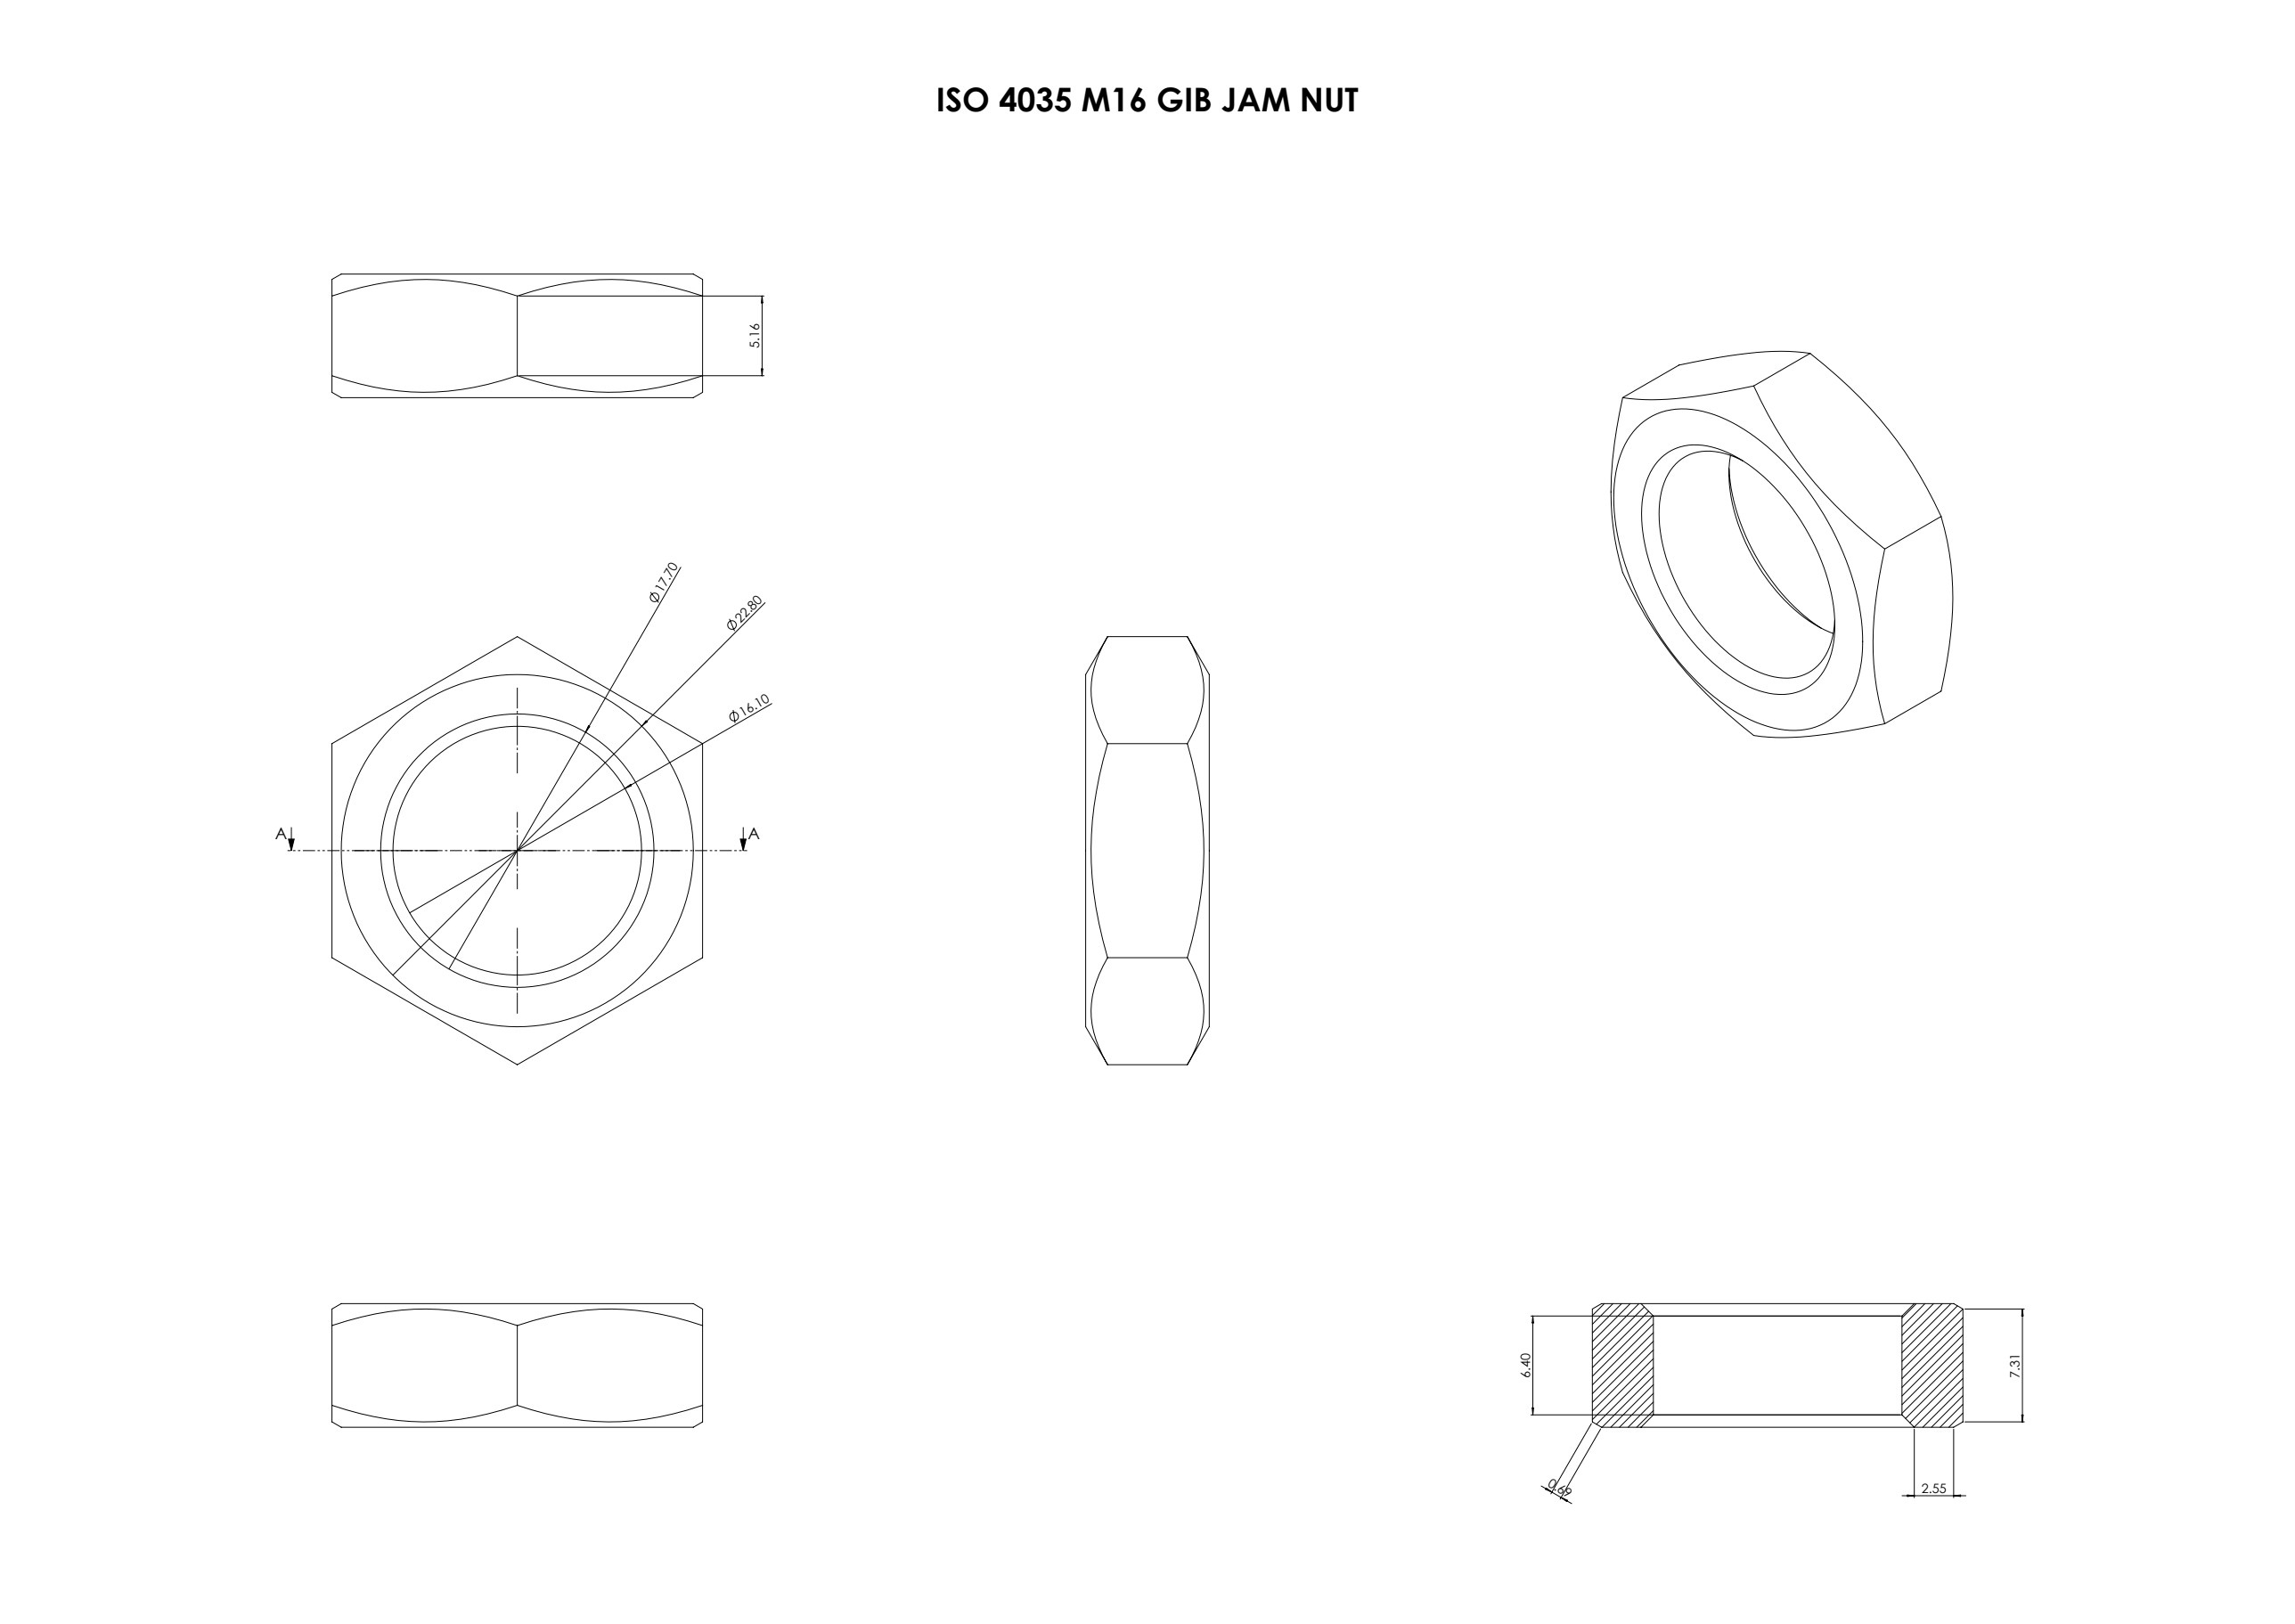
ISO-10303-21;
HEADER;
/* Generated by software containing ST-Developer
 * from STEP Tools, Inc. (www.steptools.com) 
 */

FILE_DESCRIPTION(
/* description */ (''),
/* implementation_level */ '2;1');

FILE_NAME(
/* name */ '12_ISO_4035_M16_Gib_Jam_Nut.step',
/* time_stamp */ '2026-10-19T23:58:09-07:00',
/* author */ (''),
/* organization */ (''),
/* preprocessor_version */ 'ST-DEVELOPER v20.2',
/* originating_system */ 'Autodesk Translation Framework v15.15.0.0',
/* authorisation */ '');

FILE_SCHEMA (('AP203_CONFIGURATION_CONTROLLED_3D_DESIGN_OF_MECHANICAL_PARTS_AND_ASSEMBLIES_MIM_LF { 1 0 10303 203 3 1 4 }',
'AUTOMOTIVE_DESIGN { 1 0 10303 214 3 1 1 }','INTEGRATED_CNC_SCHEMA','MODEL_BASED_INTEGRATED_MANUFACTURING_SCHEMA',
'PROCESS_PLANNING_SCHEMA','AP242_MANAGED_MODEL_BASED_3D_ENGINEERING_MIM_LF { 1 0 10303 442 3 1 4 }'));
ENDSEC;

DATA;
#10=MECHANICAL_DESIGN_GEOMETRIC_PRESENTATION_REPRESENTATION('',(#415),#70757);
#227=(
BOUNDED_CURVE()
B_SPLINE_CURVE(2,(#54642,#54643,#54644),.UNSPECIFIED.,.F.,.F.)
B_SPLINE_CURVE_WITH_KNOTS((3,3),(0.083069206448341,0.799733019594622),
 .UNSPECIFIED.)
CURVE()
GEOMETRIC_REPRESENTATION_ITEM()
RATIONAL_B_SPLINE_CURVE((1.01933756729741,1.09818360252296,1.09818360252296))
REPRESENTATION_ITEM('')
);
#228=(
BOUNDED_CURVE()
B_SPLINE_CURVE(2,(#54646,#54647,#54648),.UNSPECIFIED.,.F.,.F.)
B_SPLINE_CURVE_WITH_KNOTS((3,3),(0.0830692064483412,1.5163968327409),
 .UNSPECIFIED.)
CURVE()
GEOMETRIC_REPRESENTATION_ITEM()
RATIONAL_B_SPLINE_CURVE((1.01933756729741,1.17702963774851,1.01933756729741))
REPRESENTATION_ITEM('')
);
#229=(
BOUNDED_CURVE()
B_SPLINE_CURVE(2,(#54650,#54651,#54652),.UNSPECIFIED.,.F.,.F.)
B_SPLINE_CURVE_WITH_KNOTS((3,3),(0.0830692064483411,1.5163968327409),
 .UNSPECIFIED.)
CURVE()
GEOMETRIC_REPRESENTATION_ITEM()
RATIONAL_B_SPLINE_CURVE((1.01933756729741,1.17702963774851,1.01933756729741))
REPRESENTATION_ITEM('')
);
#230=(
BOUNDED_CURVE()
B_SPLINE_CURVE(2,(#54654,#54655,#54656),.UNSPECIFIED.,.F.,.F.)
B_SPLINE_CURVE_WITH_KNOTS((3,3),(0.0830692064483411,1.5163968327409),
 .UNSPECIFIED.)
CURVE()
GEOMETRIC_REPRESENTATION_ITEM()
RATIONAL_B_SPLINE_CURVE((1.01933756729741,1.17702963774851,1.01933756729741))
REPRESENTATION_ITEM('')
);
#231=(
BOUNDED_CURVE()
B_SPLINE_CURVE(2,(#54658,#54659,#54660),.UNSPECIFIED.,.F.,.F.)
B_SPLINE_CURVE_WITH_KNOTS((3,3),(0.083069206448341,1.5163968327409),
 .UNSPECIFIED.)
CURVE()
GEOMETRIC_REPRESENTATION_ITEM()
RATIONAL_B_SPLINE_CURVE((1.01933756729741,1.17702963774852,1.01933756729741))
REPRESENTATION_ITEM('')
);
#232=(
BOUNDED_CURVE()
B_SPLINE_CURVE(2,(#54662,#54663,#54664),.UNSPECIFIED.,.F.,.F.)
B_SPLINE_CURVE_WITH_KNOTS((3,3),(0.0830692064483414,1.5163968327409),
 .UNSPECIFIED.)
CURVE()
GEOMETRIC_REPRESENTATION_ITEM()
RATIONAL_B_SPLINE_CURVE((1.01933756729741,1.17702963774851,1.01933756729741))
REPRESENTATION_ITEM('')
);
#233=(
BOUNDED_CURVE()
B_SPLINE_CURVE(2,(#54665,#54666,#54667),.UNSPECIFIED.,.F.,.F.)
B_SPLINE_CURVE_WITH_KNOTS((3,3),(0.799733019594622,1.5163968327409),
 .UNSPECIFIED.)
CURVE()
GEOMETRIC_REPRESENTATION_ITEM()
RATIONAL_B_SPLINE_CURVE((1.09818360252296,1.09818360252296,1.01933756729741))
REPRESENTATION_ITEM('')
);
#234=(
BOUNDED_CURVE()
B_SPLINE_CURVE(2,(#54672,#54673,#54674),.UNSPECIFIED.,.F.,.F.)
B_SPLINE_CURVE_WITH_KNOTS((3,3),(0.083069206448341,1.5163968327409),
 .UNSPECIFIED.)
CURVE()
GEOMETRIC_REPRESENTATION_ITEM()
RATIONAL_B_SPLINE_CURVE((1.01933756729741,1.17702963774851,1.01933756729741))
REPRESENTATION_ITEM('')
);
#235=(
BOUNDED_CURVE()
B_SPLINE_CURVE(2,(#54679,#54680,#54681),.UNSPECIFIED.,.F.,.F.)
B_SPLINE_CURVE_WITH_KNOTS((3,3),(0.083069206448341,1.5163968327409),
 .UNSPECIFIED.)
CURVE()
GEOMETRIC_REPRESENTATION_ITEM()
RATIONAL_B_SPLINE_CURVE((1.01933756729741,1.17702963774851,1.01933756729741))
REPRESENTATION_ITEM('')
);
#236=(
BOUNDED_CURVE()
B_SPLINE_CURVE(2,(#54685,#54686,#54687),.UNSPECIFIED.,.F.,.F.)
B_SPLINE_CURVE_WITH_KNOTS((3,3),(0.0830692064483412,1.5163968327409),
 .UNSPECIFIED.)
CURVE()
GEOMETRIC_REPRESENTATION_ITEM()
RATIONAL_B_SPLINE_CURVE((1.01933756729741,1.17702963774851,1.01933756729741))
REPRESENTATION_ITEM('')
);
#237=(
BOUNDED_CURVE()
B_SPLINE_CURVE(2,(#54690,#54691,#54692),.UNSPECIFIED.,.F.,.F.)
B_SPLINE_CURVE_WITH_KNOTS((3,3),(0.0830692064483409,1.5163968327409),
 .UNSPECIFIED.)
CURVE()
GEOMETRIC_REPRESENTATION_ITEM()
RATIONAL_B_SPLINE_CURVE((1.01933756729741,1.17702963774851,1.01933756729741))
REPRESENTATION_ITEM('')
);
#238=(
BOUNDED_CURVE()
B_SPLINE_CURVE(2,(#54694,#54695,#54696),.UNSPECIFIED.,.F.,.F.)
B_SPLINE_CURVE_WITH_KNOTS((3,3),(0.799733019594622,1.5163968327409),
 .UNSPECIFIED.)
CURVE()
GEOMETRIC_REPRESENTATION_ITEM()
RATIONAL_B_SPLINE_CURVE((1.09818360252296,1.09818360252296,1.01933756729741))
REPRESENTATION_ITEM('')
);
#239=(
BOUNDED_CURVE()
B_SPLINE_CURVE(2,(#54699,#54700,#54701),.UNSPECIFIED.,.F.,.F.)
B_SPLINE_CURVE_WITH_KNOTS((3,3),(0.0830692064483412,0.799733019594622),
 .UNSPECIFIED.)
CURVE()
GEOMETRIC_REPRESENTATION_ITEM()
RATIONAL_B_SPLINE_CURVE((1.01933756729741,1.09818360252296,1.09818360252296))
REPRESENTATION_ITEM('')
);
#240=(
BOUNDED_CURVE()
B_SPLINE_CURVE(2,(#54702,#54703,#54704),.UNSPECIFIED.,.F.,.F.)
B_SPLINE_CURVE_WITH_KNOTS((3,3),(0.0830692064483414,1.5163968327409),
 .UNSPECIFIED.)
CURVE()
GEOMETRIC_REPRESENTATION_ITEM()
RATIONAL_B_SPLINE_CURVE((1.01933756729741,1.17702963774851,1.01933756729741))
REPRESENTATION_ITEM('')
);
#385=SHAPE_REPRESENTATION_RELATIONSHIP('SRR','None',#70826,#400);
#400=ADVANCED_BREP_SHAPE_REPRESENTATION('',(#475),#70750);
#415=STYLED_ITEM('',(#71054),#475);
#475=MANIFOLD_SOLID_BREP('Nut',#26880);
#682=CYLINDRICAL_SURFACE('',#27673,0.805);
#865=FACE_BOUND('',#4523,.T.);
#866=FACE_BOUND('',#4526,.T.);
#1869=PLANE('',#27675);
#1870=PLANE('',#27679);
#1871=PLANE('',#27682);
#1872=PLANE('',#27683);
#1873=PLANE('',#27684);
#1874=PLANE('',#27686);
#1875=PLANE('',#27687);
#1876=PLANE('',#27688);
#3011=FACE_OUTER_BOUND('',#4520,.T.);
#3012=FACE_OUTER_BOUND('',#4521,.T.);
#3013=FACE_OUTER_BOUND('',#4522,.T.);
#3014=FACE_OUTER_BOUND('',#4524,.T.);
#3015=FACE_OUTER_BOUND('',#4525,.T.);
#3016=FACE_OUTER_BOUND('',#4527,.T.);
#3017=FACE_OUTER_BOUND('',#4528,.T.);
#3018=FACE_OUTER_BOUND('',#4529,.T.);
#3019=FACE_OUTER_BOUND('',#4530,.T.);
#3020=FACE_OUTER_BOUND('',#4531,.T.);
#3021=FACE_OUTER_BOUND('',#4532,.T.);
#3022=FACE_OUTER_BOUND('',#4533,.T.);
#3023=FACE_OUTER_BOUND('',#4534,.T.);
#4520=EDGE_LOOP('',(#19794,#19795,#19796,#19797));
#4521=EDGE_LOOP('',(#19798,#19799,#19800,#19801));
#4522=EDGE_LOOP('',(#19802));
#4523=EDGE_LOOP('',(#19803));
#4524=EDGE_LOOP('',(#19804,#19805,#19806,#19807));
#4525=EDGE_LOOP('',(#19808));
#4526=EDGE_LOOP('',(#19809));
#4527=EDGE_LOOP('',(#19810,#19811,#19812,#19813,#19814,#19815,#19816,#19817,
#19818,#19819));
#4528=EDGE_LOOP('',(#19820,#19821,#19822,#19823));
#4529=EDGE_LOOP('',(#19824,#19825,#19826,#19827));
#4530=EDGE_LOOP('',(#19828,#19829,#19830,#19831));
#4531=EDGE_LOOP('',(#19832,#19833,#19834,#19835,#19836,#19837,#19838,#19839,
#19840,#19841));
#4532=EDGE_LOOP('',(#19842,#19843,#19844,#19845));
#4533=EDGE_LOOP('',(#19846,#19847,#19848,#19849));
#4534=EDGE_LOOP('',(#19850,#19851,#19852,#19853,#19854,#19855));
#6146=LINE('',#54622,#8643);
#6147=LINE('',#54627,#8644);
#6148=LINE('',#54634,#8645);
#6149=LINE('',#54640,#8646);
#6150=LINE('',#54670,#8647);
#6151=LINE('',#54675,#8648);
#6152=LINE('',#54678,#8649);
#6153=LINE('',#54684,#8650);
#6154=LINE('',#54697,#8651);
#6155=LINE('',#54706,#8652);
#6156=LINE('',#54708,#8653);
#8643=VECTOR('',#30739,0.845);
#8644=VECTOR('',#30746,0.805);
#8645=VECTOR('',#30755,0.845);
#8646=VECTOR('',#30762,1.28782032302755);
#8647=VECTOR('',#30765,1.);
#8648=VECTOR('',#30766,1.);
#8649=VECTOR('',#30769,1.);
#8650=VECTOR('',#30772,1.);
#8651=VECTOR('',#30775,1.28782032302755);
#8652=VECTOR('',#30778,1.);
#8653=VECTOR('',#30781,1.);
#10834=CIRCLE('',#27671,0.805);
#10835=CIRCLE('',#27672,0.885);
#10836=CIRCLE('',#27674,0.805);
#10837=CIRCLE('',#27676,1.14);
#10838=CIRCLE('',#27678,0.885);
#10839=CIRCLE('',#27680,1.14);
#11864=VERTEX_POINT('',#54619);
#11865=VERTEX_POINT('',#54621);
#11866=VERTEX_POINT('',#54625);
#11867=VERTEX_POINT('',#54629);
#11868=VERTEX_POINT('',#54632);
#11869=VERTEX_POINT('',#54636);
#11870=VERTEX_POINT('',#54639);
#11871=VERTEX_POINT('',#54641);
#11872=VERTEX_POINT('',#54645);
#11873=VERTEX_POINT('',#54649);
#11874=VERTEX_POINT('',#54653);
#11875=VERTEX_POINT('',#54657);
#11876=VERTEX_POINT('',#54661);
#11877=VERTEX_POINT('',#54669);
#11878=VERTEX_POINT('',#54671);
#11879=VERTEX_POINT('',#54677);
#11880=VERTEX_POINT('',#54683);
#11881=VERTEX_POINT('',#54689);
#11882=VERTEX_POINT('',#54693);
#11883=VERTEX_POINT('',#54698);
#14750=EDGE_CURVE('',#11864,#11864,#10834,.T.);
#14751=EDGE_CURVE('',#11864,#11865,#6146,.T.);
#14752=EDGE_CURVE('',#11865,#11865,#10835,.T.);
#14753=EDGE_CURVE('',#11866,#11866,#10836,.T.);
#14754=EDGE_CURVE('',#11866,#11864,#6147,.T.);
#14755=EDGE_CURVE('',#11867,#11867,#10837,.T.);
#14756=EDGE_CURVE('',#11868,#11868,#10838,.T.);
#14757=EDGE_CURVE('',#11868,#11866,#6148,.T.);
#14758=EDGE_CURVE('',#11869,#11869,#10839,.T.);
#14759=EDGE_CURVE('',#11867,#11870,#6149,.T.);
#14760=EDGE_CURVE('',#11871,#11870,#227,.T.);
#14761=EDGE_CURVE('',#11872,#11871,#228,.T.);
#14762=EDGE_CURVE('',#11873,#11872,#229,.T.);
#14763=EDGE_CURVE('',#11874,#11873,#230,.T.);
#14764=EDGE_CURVE('',#11875,#11874,#231,.T.);
#14765=EDGE_CURVE('',#11876,#11875,#232,.T.);
#14766=EDGE_CURVE('',#11870,#11876,#233,.T.);
#14767=EDGE_CURVE('',#11874,#11877,#6150,.T.);
#14768=EDGE_CURVE('',#11877,#11878,#234,.T.);
#14769=EDGE_CURVE('',#11875,#11878,#6151,.T.);
#14770=EDGE_CURVE('',#11873,#11879,#6152,.T.);
#14771=EDGE_CURVE('',#11879,#11877,#235,.T.);
#14772=EDGE_CURVE('',#11872,#11880,#6153,.T.);
#14773=EDGE_CURVE('',#11880,#11879,#236,.T.);
#14774=EDGE_CURVE('',#11881,#11880,#237,.T.);
#14775=EDGE_CURVE('',#11882,#11881,#238,.T.);
#14776=EDGE_CURVE('',#11882,#11869,#6154,.T.);
#14777=EDGE_CURVE('',#11883,#11882,#239,.T.);
#14778=EDGE_CURVE('',#11878,#11883,#240,.T.);
#14779=EDGE_CURVE('',#11871,#11881,#6155,.T.);
#14780=EDGE_CURVE('',#11876,#11883,#6156,.T.);
#19794=ORIENTED_EDGE('',*,*,#14750,.T.);
#19795=ORIENTED_EDGE('',*,*,#14751,.T.);
#19796=ORIENTED_EDGE('',*,*,#14752,.T.);
#19797=ORIENTED_EDGE('',*,*,#14751,.F.);
#19798=ORIENTED_EDGE('',*,*,#14753,.F.);
#19799=ORIENTED_EDGE('',*,*,#14754,.T.);
#19800=ORIENTED_EDGE('',*,*,#14750,.F.);
#19801=ORIENTED_EDGE('',*,*,#14754,.F.);
#19802=ORIENTED_EDGE('',*,*,#14755,.T.);
#19803=ORIENTED_EDGE('',*,*,#14752,.F.);
#19804=ORIENTED_EDGE('',*,*,#14756,.T.);
#19805=ORIENTED_EDGE('',*,*,#14757,.T.);
#19806=ORIENTED_EDGE('',*,*,#14753,.T.);
#19807=ORIENTED_EDGE('',*,*,#14757,.F.);
#19808=ORIENTED_EDGE('',*,*,#14758,.T.);
#19809=ORIENTED_EDGE('',*,*,#14756,.F.);
#19810=ORIENTED_EDGE('',*,*,#14755,.F.);
#19811=ORIENTED_EDGE('',*,*,#14759,.T.);
#19812=ORIENTED_EDGE('',*,*,#14760,.F.);
#19813=ORIENTED_EDGE('',*,*,#14761,.F.);
#19814=ORIENTED_EDGE('',*,*,#14762,.F.);
#19815=ORIENTED_EDGE('',*,*,#14763,.F.);
#19816=ORIENTED_EDGE('',*,*,#14764,.F.);
#19817=ORIENTED_EDGE('',*,*,#14765,.F.);
#19818=ORIENTED_EDGE('',*,*,#14766,.F.);
#19819=ORIENTED_EDGE('',*,*,#14759,.F.);
#19820=ORIENTED_EDGE('',*,*,#14764,.T.);
#19821=ORIENTED_EDGE('',*,*,#14767,.T.);
#19822=ORIENTED_EDGE('',*,*,#14768,.T.);
#19823=ORIENTED_EDGE('',*,*,#14769,.F.);
#19824=ORIENTED_EDGE('',*,*,#14763,.T.);
#19825=ORIENTED_EDGE('',*,*,#14770,.T.);
#19826=ORIENTED_EDGE('',*,*,#14771,.T.);
#19827=ORIENTED_EDGE('',*,*,#14767,.F.);
#19828=ORIENTED_EDGE('',*,*,#14762,.T.);
#19829=ORIENTED_EDGE('',*,*,#14772,.T.);
#19830=ORIENTED_EDGE('',*,*,#14773,.T.);
#19831=ORIENTED_EDGE('',*,*,#14770,.F.);
#19832=ORIENTED_EDGE('',*,*,#14768,.F.);
#19833=ORIENTED_EDGE('',*,*,#14771,.F.);
#19834=ORIENTED_EDGE('',*,*,#14773,.F.);
#19835=ORIENTED_EDGE('',*,*,#14774,.F.);
#19836=ORIENTED_EDGE('',*,*,#14775,.F.);
#19837=ORIENTED_EDGE('',*,*,#14776,.T.);
#19838=ORIENTED_EDGE('',*,*,#14758,.F.);
#19839=ORIENTED_EDGE('',*,*,#14776,.F.);
#19840=ORIENTED_EDGE('',*,*,#14777,.F.);
#19841=ORIENTED_EDGE('',*,*,#14778,.F.);
#19842=ORIENTED_EDGE('',*,*,#14761,.T.);
#19843=ORIENTED_EDGE('',*,*,#14779,.T.);
#19844=ORIENTED_EDGE('',*,*,#14774,.T.);
#19845=ORIENTED_EDGE('',*,*,#14772,.F.);
#19846=ORIENTED_EDGE('',*,*,#14765,.T.);
#19847=ORIENTED_EDGE('',*,*,#14769,.T.);
#19848=ORIENTED_EDGE('',*,*,#14778,.T.);
#19849=ORIENTED_EDGE('',*,*,#14780,.F.);
#19850=ORIENTED_EDGE('',*,*,#14760,.T.);
#19851=ORIENTED_EDGE('',*,*,#14766,.T.);
#19852=ORIENTED_EDGE('',*,*,#14780,.T.);
#19853=ORIENTED_EDGE('',*,*,#14777,.T.);
#19854=ORIENTED_EDGE('',*,*,#14775,.T.);
#19855=ORIENTED_EDGE('',*,*,#14779,.F.);
#25333=CONICAL_SURFACE('',#27670,0.845,0.785398163397448);
#25334=CONICAL_SURFACE('',#27677,0.845,0.785398163397448);
#25335=CONICAL_SURFACE('',#27681,1.28782032302755,1.0471975511966);
#25336=CONICAL_SURFACE('',#27685,1.28782032302755,1.0471975511966);
#25824=ADVANCED_FACE('',(#3011),#25333,.F.);
#25825=ADVANCED_FACE('',(#3012),#682,.F.);
#25826=ADVANCED_FACE('',(#3013,#865),#1869,.F.);
#25827=ADVANCED_FACE('',(#3014),#25334,.F.);
#25828=ADVANCED_FACE('',(#3015,#866),#1870,.T.);
#25829=ADVANCED_FACE('',(#3016),#25335,.T.);
#25830=ADVANCED_FACE('',(#3017),#1871,.T.);
#25831=ADVANCED_FACE('',(#3018),#1872,.T.);
#25832=ADVANCED_FACE('',(#3019),#1873,.T.);
#25833=ADVANCED_FACE('',(#3020),#25336,.T.);
#25834=ADVANCED_FACE('',(#3021),#1874,.T.);
#25835=ADVANCED_FACE('',(#3022),#1875,.T.);
#25836=ADVANCED_FACE('',(#3023),#1876,.T.);
#26880=CLOSED_SHELL('',(#25824,#25825,#25826,#25827,#25828,#25829,#25830,
#25831,#25832,#25833,#25834,#25835,#25836));
#27669=AXIS2_PLACEMENT_3D('',#54617,#30733,#30734);
#27670=AXIS2_PLACEMENT_3D('',#54618,#30735,#30736);
#27671=AXIS2_PLACEMENT_3D('',#54620,#30737,#30738);
#27672=AXIS2_PLACEMENT_3D('',#54623,#30740,#30741);
#27673=AXIS2_PLACEMENT_3D('',#54624,#30742,#30743);
#27674=AXIS2_PLACEMENT_3D('',#54626,#30744,#30745);
#27675=AXIS2_PLACEMENT_3D('',#54628,#30747,#30748);
#27676=AXIS2_PLACEMENT_3D('',#54630,#30749,#30750);
#27677=AXIS2_PLACEMENT_3D('',#54631,#30751,#30752);
#27678=AXIS2_PLACEMENT_3D('',#54633,#30753,#30754);
#27679=AXIS2_PLACEMENT_3D('',#54635,#30756,#30757);
#27680=AXIS2_PLACEMENT_3D('',#54637,#30758,#30759);
#27681=AXIS2_PLACEMENT_3D('',#54638,#30760,#30761);
#27682=AXIS2_PLACEMENT_3D('',#54668,#30763,#30764);
#27683=AXIS2_PLACEMENT_3D('',#54676,#30767,#30768);
#27684=AXIS2_PLACEMENT_3D('',#54682,#30770,#30771);
#27685=AXIS2_PLACEMENT_3D('',#54688,#30773,#30774);
#27686=AXIS2_PLACEMENT_3D('',#54705,#30776,#30777);
#27687=AXIS2_PLACEMENT_3D('',#54707,#30779,#30780);
#27688=AXIS2_PLACEMENT_3D('',#54709,#30782,#30783);
#30733=DIRECTION('axis',(0.,0.,1.));
#30734=DIRECTION('refdir',(1.,0.,0.));
#30735=DIRECTION('center_axis',(0.,0.,-1.));
#30736=DIRECTION('ref_axis',(1.,0.,0.));
#30737=DIRECTION('center_axis',(0.,0.,1.));
#30738=DIRECTION('ref_axis',(1.,0.,0.));
#30739=DIRECTION('',(-0.707106781186547,-8.65956056235493E-17,-0.707106781186548));
#30740=DIRECTION('center_axis',(0.,0.,-1.));
#30741=DIRECTION('ref_axis',(1.,0.,0.));
#30742=DIRECTION('center_axis',(0.,0.,1.));
#30743=DIRECTION('ref_axis',(1.,0.,0.));
#30744=DIRECTION('center_axis',(0.,0.,-1.));
#30745=DIRECTION('ref_axis',(1.,0.,0.));
#30746=DIRECTION('',(0.,0.,-1.));
#30747=DIRECTION('center_axis',(0.,0.,1.));
#30748=DIRECTION('ref_axis',(1.,0.,0.));
#30749=DIRECTION('center_axis',(0.,0.,-1.));
#30750=DIRECTION('ref_axis',(1.,0.,0.));
#30751=DIRECTION('center_axis',(0.,0.,1.));
#30752=DIRECTION('ref_axis',(1.,0.,0.));
#30753=DIRECTION('center_axis',(0.,0.,1.));
#30754=DIRECTION('ref_axis',(1.,0.,0.));
#30755=DIRECTION('',(0.707106781186547,8.65956056235493E-17,-0.707106781186548));
#30756=DIRECTION('center_axis',(0.,0.,1.));
#30757=DIRECTION('ref_axis',(1.,0.,0.));
#30758=DIRECTION('center_axis',(0.,0.,1.));
#30759=DIRECTION('ref_axis',(1.,0.,0.));
#30760=DIRECTION('center_axis',(0.,0.,1.));
#30761=DIRECTION('ref_axis',(1.,0.,0.));
#30762=DIRECTION('',(-0.866025403784439,-1.06057523872491E-16,0.5));
#30763=DIRECTION('center_axis',(0.5,-0.866025403784439,0.));
#30764=DIRECTION('ref_axis',(0.866025403784439,0.5,0.));
#30765=DIRECTION('',(0.,0.,1.));
#30766=DIRECTION('',(0.,0.,1.));
#30767=DIRECTION('center_axis',(1.,-3.20493781063927E-16,0.));
#30768=DIRECTION('ref_axis',(3.20493781063927E-16,1.,0.));
#30769=DIRECTION('',(0.,0.,1.));
#30770=DIRECTION('center_axis',(0.5,0.866025403784439,0.));
#30771=DIRECTION('ref_axis',(-0.866025403784439,0.5,0.));
#30772=DIRECTION('',(0.,0.,1.));
#30773=DIRECTION('center_axis',(0.,0.,-1.));
#30774=DIRECTION('ref_axis',(1.,0.,0.));
#30775=DIRECTION('',(0.866025403784439,1.06057523872491E-16,0.5));
#30776=DIRECTION('center_axis',(-0.5,0.866025403784439,0.));
#30777=DIRECTION('ref_axis',(-0.866025403784439,-0.5,0.));
#30778=DIRECTION('',(0.,0.,1.));
#30779=DIRECTION('center_axis',(-0.5,-0.866025403784439,0.));
#30780=DIRECTION('ref_axis',(0.866025403784439,-0.5,0.));
#30781=DIRECTION('',(0.,0.,1.));
#30782=DIRECTION('center_axis',(-1.,-1.60246890531964E-16,0.));
#30783=DIRECTION('ref_axis',(1.60246890531964E-16,-1.,0.));
#54617=CARTESIAN_POINT('',(0.,0.,0.));
#54618=CARTESIAN_POINT('Origin',(0.,0.,0.04));
#54619=CARTESIAN_POINT('',(-0.805,-9.85840673313619E-17,0.08));
#54620=CARTESIAN_POINT('Origin',(0.,0.,0.08));
#54621=CARTESIAN_POINT('',(-0.885,1.08381241724541E-16,0.));
#54622=CARTESIAN_POINT('',(-0.845,-1.03482654527951E-16,0.04));
#54623=CARTESIAN_POINT('Origin',(0.,0.,0.));
#54624=CARTESIAN_POINT('Origin',(0.,0.,0.));
#54625=CARTESIAN_POINT('',(-0.805,9.85840673313619E-17,0.72));
#54626=CARTESIAN_POINT('Origin',(0.,0.,0.72));
#54627=CARTESIAN_POINT('',(-0.805,-9.85840673313619E-17,0.));
#54628=CARTESIAN_POINT('Origin',(0.,0.,0.));
#54629=CARTESIAN_POINT('',(-1.14,-1.39609735102798E-16,-8.32667268468867E-17));
#54630=CARTESIAN_POINT('Origin',(0.,0.,0.));
#54631=CARTESIAN_POINT('Origin',(0.,0.,0.76));
#54632=CARTESIAN_POINT('',(-0.885,-1.08381241724541E-16,0.8));
#54633=CARTESIAN_POINT('Origin',(0.,0.,0.8));
#54634=CARTESIAN_POINT('',(-0.845,-1.03482654527951E-16,0.76));
#54635=CARTESIAN_POINT('Origin',(0.,0.,0.8));
#54636=CARTESIAN_POINT('',(-1.14,-1.39609735102798E-16,0.8));
#54637=CARTESIAN_POINT('Origin',(0.,0.,0.8));
#54638=CARTESIAN_POINT('Origin',(0.,0.,0.085344103291654));
#54639=CARTESIAN_POINT('',(-1.2,-1.36663997456004E-16,0.0346410161513778));
#54640=CARTESIAN_POINT('',(-1.28782032302755,-1.5771250364726E-16,0.085344103291654));
#54641=CARTESIAN_POINT('',(-1.2,0.692820323027551,0.141820693123827));
#54642=CARTESIAN_POINT('Ctrl Pts',(-1.2,0.692820323027551,0.141820693123827));
#54643=CARTESIAN_POINT('Ctrl Pts',(-1.2,0.321539030917347,0.0346410161513777));
#54644=CARTESIAN_POINT('Ctrl Pts',(-1.2,-1.26370379014326E-16,0.0346410161513778));
#54645=CARTESIAN_POINT('',(8.48460190979925E-17,1.3856406460551,0.141820693123827));
#54646=CARTESIAN_POINT('Ctrl Pts',(8.48460190979925E-17,1.3856406460551,
0.141820693123827));
#54647=CARTESIAN_POINT('Ctrl Pts',(-0.599999999999999,1.03923048454133,
-0.0581793068761738));
#54648=CARTESIAN_POINT('Ctrl Pts',(-1.2,0.692820323027551,0.141820693123827));
#54649=CARTESIAN_POINT('',(1.2,0.692820323027551,0.141820693123827));
#54650=CARTESIAN_POINT('Ctrl Pts',(1.2,0.692820323027551,0.141820693123827));
#54651=CARTESIAN_POINT('Ctrl Pts',(0.6,1.03923048454133,-0.0581793068761734));
#54652=CARTESIAN_POINT('Ctrl Pts',(8.48460190979925E-17,1.3856406460551,
0.141820693123827));
#54653=CARTESIAN_POINT('',(1.2,-0.692820323027552,0.141820693123827));
#54654=CARTESIAN_POINT('Ctrl Pts',(1.2,-0.692820323027552,0.141820693123827));
#54655=CARTESIAN_POINT('Ctrl Pts',(1.2,-9.99200722162641E-16,-0.0581793068761738));
#54656=CARTESIAN_POINT('Ctrl Pts',(1.2,0.692820323027551,0.141820693123827));
#54657=CARTESIAN_POINT('',(-2.54538057293978E-16,-1.3856406460551,0.141820693123827));
#54658=CARTESIAN_POINT('Ctrl Pts',(-2.54538057293978E-16,-1.3856406460551,
0.141820693123827));
#54659=CARTESIAN_POINT('Ctrl Pts',(0.6,-1.03923048454133,-0.0581793068761735));
#54660=CARTESIAN_POINT('Ctrl Pts',(1.2,-0.692820323027551,0.141820693123827));
#54661=CARTESIAN_POINT('',(-1.2,-0.692820323027551,0.141820693123827));
#54662=CARTESIAN_POINT('Ctrl Pts',(-1.2,-0.692820323027551,0.141820693123827));
#54663=CARTESIAN_POINT('Ctrl Pts',(-0.6,-1.03923048454133,-0.0581793068761732));
#54664=CARTESIAN_POINT('Ctrl Pts',(-2.54538057293978E-16,-1.3856406460551,
0.141820693123827));
#54665=CARTESIAN_POINT('Ctrl Pts',(-1.2,-1.26370379014326E-16,0.0346410161513778));
#54666=CARTESIAN_POINT('Ctrl Pts',(-1.2,-0.321539030917348,0.0346410161513778));
#54667=CARTESIAN_POINT('Ctrl Pts',(-1.2,-0.692820323027551,0.141820693123827));
#54668=CARTESIAN_POINT('Origin',(-2.54538057293978E-16,-1.3856406460551,
0.));
#54669=CARTESIAN_POINT('',(1.2,-0.692820323027552,0.658179306876173));
#54670=CARTESIAN_POINT('',(1.2,-0.692820323027552,0.));
#54671=CARTESIAN_POINT('',(-2.54538057293978E-16,-1.3856406460551,0.658179306876173));
#54672=CARTESIAN_POINT('Ctrl Pts',(1.2,-0.692820323027552,0.658179306876173));
#54673=CARTESIAN_POINT('Ctrl Pts',(0.6,-1.03923048454133,0.858179306876173));
#54674=CARTESIAN_POINT('Ctrl Pts',(-2.54538057293978E-16,-1.3856406460551,
0.658179306876173));
#54675=CARTESIAN_POINT('',(-2.54538057293978E-16,-1.3856406460551,0.));
#54676=CARTESIAN_POINT('Origin',(1.2,-0.692820323027552,0.));
#54677=CARTESIAN_POINT('',(1.2,0.692820323027551,0.658179306876173));
#54678=CARTESIAN_POINT('',(1.2,0.692820323027551,0.));
#54679=CARTESIAN_POINT('Ctrl Pts',(1.2,0.692820323027551,0.658179306876173));
#54680=CARTESIAN_POINT('Ctrl Pts',(1.2,-3.33066907387547E-16,0.858179306876173));
#54681=CARTESIAN_POINT('Ctrl Pts',(1.2,-0.692820323027552,0.658179306876173));
#54682=CARTESIAN_POINT('Origin',(1.2,0.692820323027551,0.));
#54683=CARTESIAN_POINT('',(8.48460190979925E-17,1.3856406460551,0.658179306876173));
#54684=CARTESIAN_POINT('',(8.48460190979926E-17,1.3856406460551,0.));
#54685=CARTESIAN_POINT('Ctrl Pts',(8.48460190979925E-17,1.3856406460551,
0.658179306876173));
#54686=CARTESIAN_POINT('Ctrl Pts',(0.6,1.03923048454133,0.858179306876174));
#54687=CARTESIAN_POINT('Ctrl Pts',(1.2,0.692820323027551,0.658179306876173));
#54688=CARTESIAN_POINT('Origin',(0.,0.,0.714655896708346));
#54689=CARTESIAN_POINT('',(-1.2,0.692820323027551,0.658179306876173));
#54690=CARTESIAN_POINT('Ctrl Pts',(-1.2,0.692820323027551,0.658179306876173));
#54691=CARTESIAN_POINT('Ctrl Pts',(-0.6,1.03923048454133,0.858179306876173));
#54692=CARTESIAN_POINT('Ctrl Pts',(8.48460190979925E-17,1.3856406460551,
0.658179306876173));
#54693=CARTESIAN_POINT('',(-1.2,-2.29306563431106E-17,0.765358983848622));
#54694=CARTESIAN_POINT('Ctrl Pts',(-1.2,1.01096303211461E-16,0.765358983848622));
#54695=CARTESIAN_POINT('Ctrl Pts',(-1.2,0.321539030917348,0.765358983848622));
#54696=CARTESIAN_POINT('Ctrl Pts',(-1.2,0.692820323027551,0.658179306876173));
#54697=CARTESIAN_POINT('',(-1.28782032302755,-1.5771250364726E-16,0.714655896708346));
#54698=CARTESIAN_POINT('',(-1.2,-0.692820323027551,0.658179306876173));
#54699=CARTESIAN_POINT('Ctrl Pts',(-1.2,-0.692820323027551,0.658179306876173));
#54700=CARTESIAN_POINT('Ctrl Pts',(-1.2,-0.321539030917348,0.765358983848622));
#54701=CARTESIAN_POINT('Ctrl Pts',(-1.2,1.01096303211461E-16,0.765358983848622));
#54702=CARTESIAN_POINT('Ctrl Pts',(-2.54538057293978E-16,-1.3856406460551,
0.658179306876173));
#54703=CARTESIAN_POINT('Ctrl Pts',(-0.6,-1.03923048454133,0.858179306876173));
#54704=CARTESIAN_POINT('Ctrl Pts',(-1.2,-0.692820323027551,0.658179306876173));
#54705=CARTESIAN_POINT('Origin',(8.48460190979926E-17,1.3856406460551,0.));
#54706=CARTESIAN_POINT('',(-1.2,0.692820323027551,0.));
#54707=CARTESIAN_POINT('Origin',(-1.2,-0.692820323027551,0.));
#54708=CARTESIAN_POINT('',(-1.2,-0.692820323027551,0.));
#54709=CARTESIAN_POINT('Origin',(-1.2,0.692820323027551,0.));
#70733=UNCERTAINTY_MEASURE_WITH_UNIT(LENGTH_MEASURE(0.001),#70758,
'DISTANCE_ACCURACY_VALUE',
'Maximum model space distance between geometric entities at asserted c
onnectivities');
#70740=UNCERTAINTY_MEASURE_WITH_UNIT(LENGTH_MEASURE(0.001),#70758,
'DISTANCE_ACCURACY_VALUE',
'Maximum model space distance between geometric entities at asserted c
onnectivities');
#70750=(
GEOMETRIC_REPRESENTATION_CONTEXT(3)
GLOBAL_UNCERTAINTY_ASSIGNED_CONTEXT((#70733))
GLOBAL_UNIT_ASSIGNED_CONTEXT((#70758,#70760,#70761))
REPRESENTATION_CONTEXT('','3D')
);
#70757=(
GEOMETRIC_REPRESENTATION_CONTEXT(3)
GLOBAL_UNCERTAINTY_ASSIGNED_CONTEXT((#70740))
GLOBAL_UNIT_ASSIGNED_CONTEXT((#70758,#70760,#70761))
REPRESENTATION_CONTEXT('','3D')
);
#70758=(
LENGTH_UNIT()
NAMED_UNIT(*)
SI_UNIT(.CENTI.,.METRE.)
);
#70760=(
NAMED_UNIT(*)
PLANE_ANGLE_UNIT()
SI_UNIT($,.RADIAN.)
);
#70761=(
NAMED_UNIT(*)
SI_UNIT($,.STERADIAN.)
SOLID_ANGLE_UNIT()
);
#70771=SHAPE_DEFINITION_REPRESENTATION(#70787,#70826);
#70787=PRODUCT_DEFINITION_SHAPE('',$,#70843);
#70826=SHAPE_REPRESENTATION('',(#27669),#70750);
#70833=PRODUCT_DEFINITION_CONTEXT('part definition',#70883,'design');
#70843=PRODUCT_DEFINITION('2026-10-19-02-55-58-451',
'12_ISO_4035_M16_Gib_Jam_Nut',#70859,#70833);
#70859=PRODUCT_DEFINITION_FORMATION('',$,#70894);
#70883=APPLICATION_CONTEXT(
'Core Data for Automotive Mechanical Design Process');
#70884=PRODUCT_CONTEXT('part definition',#70883,'mechanical');
#70894=PRODUCT('2026-10-19-02-55-58-451','12_ISO_4035_M16_Gib_Jam_Nut',
$,(#70884));
#71048=COLOUR_RGB('Black',0.12,0.14,0.17);
#71049=FILL_AREA_STYLE_COLOUR('',#71048);
#71050=FILL_AREA_STYLE('',(#71049));
#71051=SURFACE_STYLE_FILL_AREA(#71050);
#71052=SURFACE_SIDE_STYLE('',(#71051));
#71053=SURFACE_STYLE_USAGE(.BOTH.,#71052);
#71054=PRESENTATION_STYLE_ASSIGNMENT((#71053));
ENDSEC;
END-ISO-10303-21;
